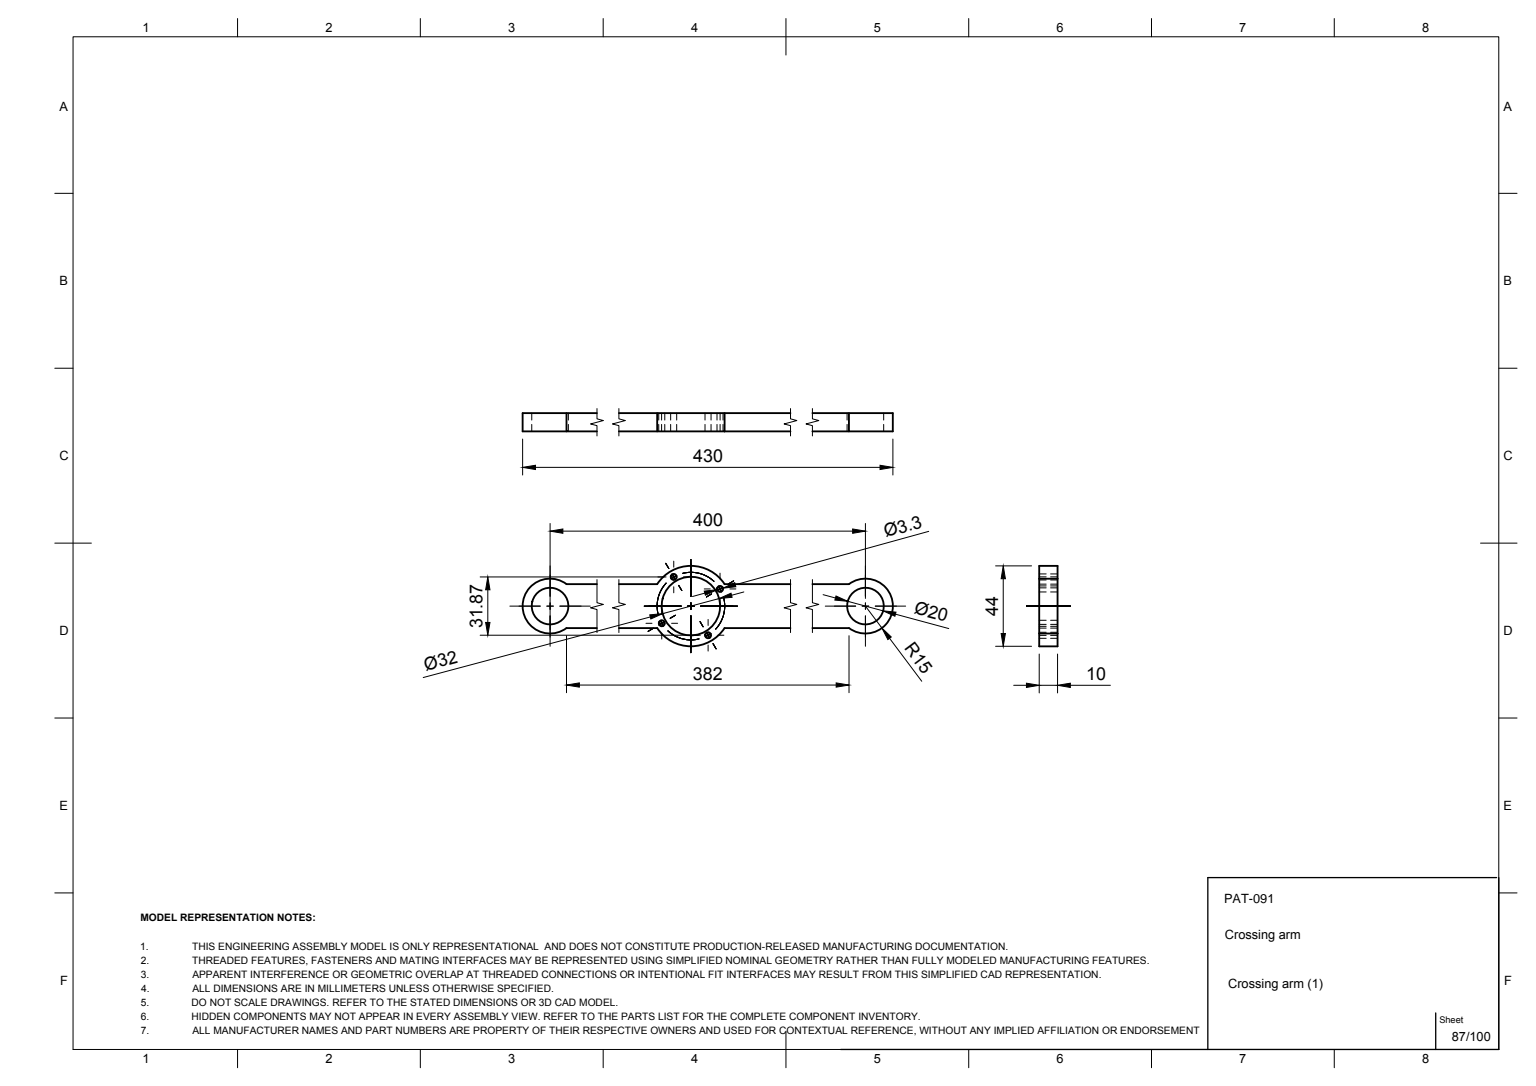
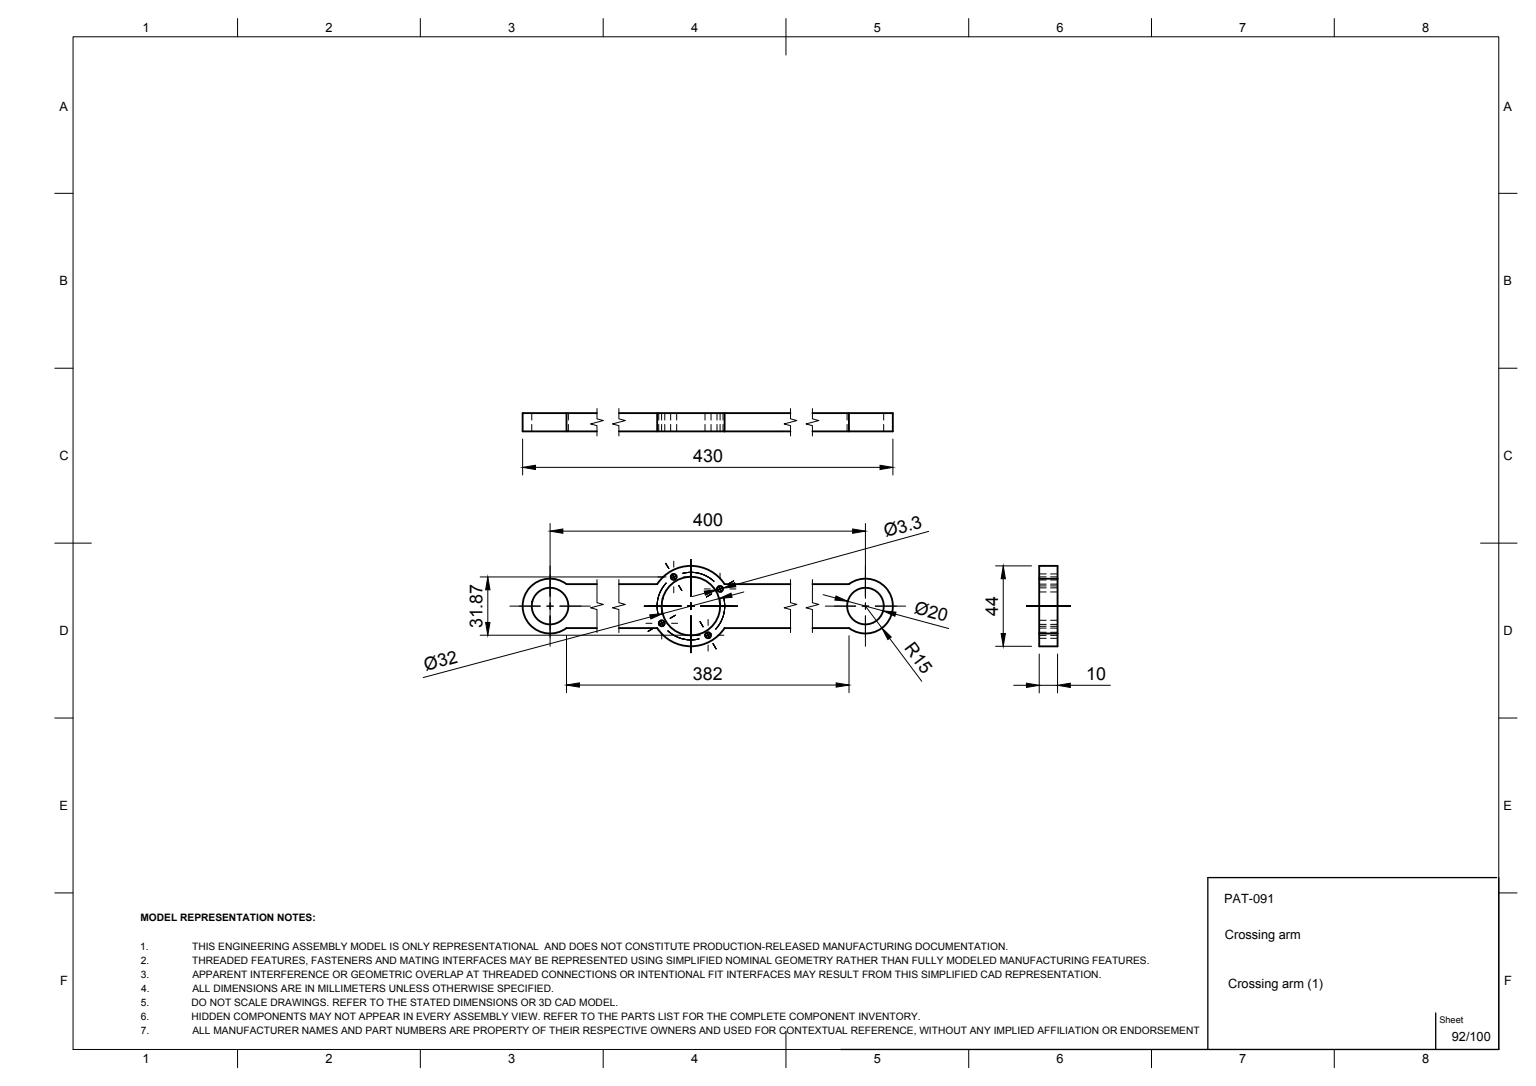
ISO-10303-21;
HEADER;
/* Generated by software containing ST-Developer
 * from STEP Tools, Inc. (www.steptools.com) 
 */

FILE_DESCRIPTION(
/* description */ ('PAT-091'),
/* implementation_level */ '2;1');

FILE_NAME(
/* name */ 'Crossing arm (1).step',
/* time_stamp */ '2026-10-27T15:34:44-07:00',
/* author */ (''),
/* organization */ (''),
/* preprocessor_version */ 'ST-DEVELOPER v20.2',
/* originating_system */ 'Autodesk Translation Framework v15.17.0.0',
/* authorisation */ '');

FILE_SCHEMA (('AUTOMOTIVE_DESIGN { 1 0 10303 214 3 1 1 }'));
ENDSEC;

DATA;
#10=MECHANICAL_DESIGN_GEOMETRIC_PRESENTATION_REPRESENTATION('',(#1057),#25100);
#837=SHAPE_REPRESENTATION_RELATIONSHIP('SRR','None',#25604,#947);
#947=ADVANCED_BREP_SHAPE_REPRESENTATION('',(#1178),#25074);
#1057=STYLED_ITEM('',(#26177),#1178);
#1178=MANIFOLD_SOLID_BREP('Body1',#13337);
#1571=FACE_BOUND('',#3877,.T.);
#1572=FACE_BOUND('',#3878,.T.);
#1573=FACE_BOUND('',#3879,.T.);
#1574=FACE_BOUND('',#3880,.T.);
#1575=FACE_BOUND('',#3881,.T.);
#1576=FACE_BOUND('',#3882,.T.);
#1577=FACE_BOUND('',#3883,.T.);
#1578=FACE_BOUND('',#3892,.T.);
#1579=FACE_BOUND('',#3893,.T.);
#1580=FACE_BOUND('',#3894,.T.);
#1581=FACE_BOUND('',#3895,.T.);
#1582=FACE_BOUND('',#3896,.T.);
#1583=FACE_BOUND('',#3897,.T.);
#1584=FACE_BOUND('',#3898,.T.);
#1986=PLANE('',#15974);
#1987=PLANE('',#15975);
#1988=PLANE('',#15980);
#1989=PLANE('',#15985);
#1990=PLANE('',#15990);
#1991=PLANE('',#15991);
#2694=FACE_OUTER_BOUND('',#3868,.T.);
#2695=FACE_OUTER_BOUND('',#3869,.T.);
#2696=FACE_OUTER_BOUND('',#3870,.T.);
#2697=FACE_OUTER_BOUND('',#3871,.T.);
#2698=FACE_OUTER_BOUND('',#3872,.T.);
#2699=FACE_OUTER_BOUND('',#3873,.T.);
#2700=FACE_OUTER_BOUND('',#3874,.T.);
#2701=FACE_OUTER_BOUND('',#3875,.T.);
#2702=FACE_OUTER_BOUND('',#3876,.T.);
#2703=FACE_OUTER_BOUND('',#3884,.T.);
#2704=FACE_OUTER_BOUND('',#3885,.T.);
#2705=FACE_OUTER_BOUND('',#3886,.T.);
#2706=FACE_OUTER_BOUND('',#3887,.T.);
#2707=FACE_OUTER_BOUND('',#3888,.T.);
#2708=FACE_OUTER_BOUND('',#3889,.T.);
#2709=FACE_OUTER_BOUND('',#3890,.T.);
#2710=FACE_OUTER_BOUND('',#3891,.T.);
#3868=EDGE_LOOP('',(#11426,#11427,#11428,#11429));
#3869=EDGE_LOOP('',(#11430,#11431,#11432,#11433));
#3870=EDGE_LOOP('',(#11434,#11435,#11436,#11437));
#3871=EDGE_LOOP('',(#11438,#11439,#11440,#11441));
#3872=EDGE_LOOP('',(#11442,#11443,#11444,#11445));
#3873=EDGE_LOOP('',(#11446,#11447,#11448,#11449));
#3874=EDGE_LOOP('',(#11450,#11451,#11452,#11453));
#3875=EDGE_LOOP('',(#11454,#11455,#11456,#11457));
#3876=EDGE_LOOP('',(#11458,#11459,#11460,#11461,#11462,#11463,#11464,#11465));
#3877=EDGE_LOOP('',(#11466));
#3878=EDGE_LOOP('',(#11467));
#3879=EDGE_LOOP('',(#11468));
#3880=EDGE_LOOP('',(#11469));
#3881=EDGE_LOOP('',(#11470));
#3882=EDGE_LOOP('',(#11471));
#3883=EDGE_LOOP('',(#11472));
#3884=EDGE_LOOP('',(#11473,#11474,#11475,#11476));
#3885=EDGE_LOOP('',(#11477,#11478,#11479,#11480));
#3886=EDGE_LOOP('',(#11481,#11482,#11483,#11484));
#3887=EDGE_LOOP('',(#11485,#11486,#11487,#11488));
#3888=EDGE_LOOP('',(#11489,#11490,#11491,#11492));
#3889=EDGE_LOOP('',(#11493,#11494,#11495,#11496));
#3890=EDGE_LOOP('',(#11497,#11498,#11499,#11500));
#3891=EDGE_LOOP('',(#11501,#11502,#11503,#11504,#11505,#11506,#11507,#11508));
#3892=EDGE_LOOP('',(#11509));
#3893=EDGE_LOOP('',(#11510));
#3894=EDGE_LOOP('',(#11511));
#3895=EDGE_LOOP('',(#11512));
#3896=EDGE_LOOP('',(#11513));
#3897=EDGE_LOOP('',(#11514));
#3898=EDGE_LOOP('',(#11515));
#4779=LINE('',#23871,#5519);
#4780=LINE('',#23877,#5520);
#4781=LINE('',#23883,#5521);
#4782=LINE('',#23889,#5522);
#4783=LINE('',#23895,#5523);
#4784=LINE('',#23900,#5524);
#4785=LINE('',#23904,#5525);
#4786=LINE('',#23909,#5526);
#4787=LINE('',#23913,#5527);
#4788=LINE('',#23917,#5528);
#4789=LINE('',#23919,#5529);
#4790=LINE('',#23920,#5530);
#4791=LINE('',#23924,#5531);
#4792=LINE('',#23926,#5532);
#4793=LINE('',#23929,#5533);
#4794=LINE('',#23936,#5534);
#4795=LINE('',#23937,#5535);
#4796=LINE('',#23941,#5536);
#4797=LINE('',#23944,#5537);
#4798=LINE('',#23947,#5538);
#4799=LINE('',#23949,#5539);
#4800=LINE('',#23953,#5540);
#4801=LINE('',#23957,#5541);
#5519=VECTOR('',#19863,0.164999999999999);
#5520=VECTOR('',#19870,0.164999999999999);
#5521=VECTOR('',#19877,0.164999999999999);
#5522=VECTOR('',#19884,0.164999999999999);
#5523=VECTOR('',#19891,1.6);
#5524=VECTOR('',#19896,1.);
#5525=VECTOR('',#19899,1.);
#5526=VECTOR('',#19904,1.);
#5527=VECTOR('',#19907,1.);
#5528=VECTOR('',#19912,1.);
#5529=VECTOR('',#19913,1.);
#5530=VECTOR('',#19914,1.);
#5531=VECTOR('',#19919,1.);
#5532=VECTOR('',#19920,1.);
#5533=VECTOR('',#19923,1.);
#5534=VECTOR('',#19930,1.);
#5535=VECTOR('',#19931,1.);
#5536=VECTOR('',#19936,1.);
#5537=VECTOR('',#19939,1.);
#5538=VECTOR('',#19942,1.);
#5539=VECTOR('',#19945,1.);
#5540=VECTOR('',#19950,1.);
#5541=VECTOR('',#19957,1.);
#6172=CIRCLE('',#15954,0.164999999999999);
#6173=CIRCLE('',#15955,0.164999999999999);
#6174=CIRCLE('',#15957,0.164999999999999);
#6175=CIRCLE('',#15958,0.164999999999999);
#6176=CIRCLE('',#15960,0.164999999999999);
#6177=CIRCLE('',#15961,0.164999999999999);
#6178=CIRCLE('',#15963,0.164999999999999);
#6179=CIRCLE('',#15964,0.164999999999999);
#6180=CIRCLE('',#15966,1.6);
#6181=CIRCLE('',#15967,1.6);
#6182=CIRCLE('',#15969,2.2);
#6183=CIRCLE('',#15970,2.2);
#6184=CIRCLE('',#15972,2.2);
#6185=CIRCLE('',#15973,2.2);
#6186=CIRCLE('',#15976,1.5);
#6187=CIRCLE('',#15977,1.5);
#6188=CIRCLE('',#15978,1.);
#6189=CIRCLE('',#15979,1.);
#6190=CIRCLE('',#15982,1.);
#6191=CIRCLE('',#15984,1.5);
#6192=CIRCLE('',#15987,1.);
#6193=CIRCLE('',#15989,1.5);
#7197=VERTEX_POINT('',#23868);
#7198=VERTEX_POINT('',#23870);
#7199=VERTEX_POINT('',#23874);
#7200=VERTEX_POINT('',#23876);
#7201=VERTEX_POINT('',#23880);
#7202=VERTEX_POINT('',#23882);
#7203=VERTEX_POINT('',#23886);
#7204=VERTEX_POINT('',#23888);
#7205=VERTEX_POINT('',#23892);
#7206=VERTEX_POINT('',#23894);
#7207=VERTEX_POINT('',#23898);
#7208=VERTEX_POINT('',#23899);
#7209=VERTEX_POINT('',#23901);
#7210=VERTEX_POINT('',#23903);
#7211=VERTEX_POINT('',#23907);
#7212=VERTEX_POINT('',#23908);
#7213=VERTEX_POINT('',#23910);
#7214=VERTEX_POINT('',#23912);
#7215=VERTEX_POINT('',#23916);
#7216=VERTEX_POINT('',#23918);
#7217=VERTEX_POINT('',#23922);
#7218=VERTEX_POINT('',#23925);
#7219=VERTEX_POINT('',#23927);
#7220=VERTEX_POINT('',#23930);
#7221=VERTEX_POINT('',#23932);
#7222=VERTEX_POINT('',#23935);
#7223=VERTEX_POINT('',#23939);
#7224=VERTEX_POINT('',#23943);
#7225=VERTEX_POINT('',#23945);
#7226=VERTEX_POINT('',#23951);
#8648=EDGE_CURVE('',#7197,#7197,#6172,.T.);
#8649=EDGE_CURVE('',#7197,#7198,#4779,.T.);
#8650=EDGE_CURVE('',#7198,#7198,#6173,.T.);
#8651=EDGE_CURVE('',#7199,#7199,#6174,.T.);
#8652=EDGE_CURVE('',#7199,#7200,#4780,.T.);
#8653=EDGE_CURVE('',#7200,#7200,#6175,.T.);
#8654=EDGE_CURVE('',#7201,#7201,#6176,.T.);
#8655=EDGE_CURVE('',#7201,#7202,#4781,.T.);
#8656=EDGE_CURVE('',#7202,#7202,#6177,.T.);
#8657=EDGE_CURVE('',#7203,#7203,#6178,.T.);
#8658=EDGE_CURVE('',#7203,#7204,#4782,.T.);
#8659=EDGE_CURVE('',#7204,#7204,#6179,.T.);
#8660=EDGE_CURVE('',#7205,#7205,#6180,.T.);
#8661=EDGE_CURVE('',#7205,#7206,#4783,.T.);
#8662=EDGE_CURVE('',#7206,#7206,#6181,.T.);
#8663=EDGE_CURVE('',#7207,#7208,#4784,.T.);
#8664=EDGE_CURVE('',#7209,#7207,#6182,.T.);
#8665=EDGE_CURVE('',#7210,#7209,#4785,.T.);
#8666=EDGE_CURVE('',#7210,#7208,#6183,.T.);
#8667=EDGE_CURVE('',#7211,#7212,#4786,.T.);
#8668=EDGE_CURVE('',#7211,#7213,#6184,.T.);
#8669=EDGE_CURVE('',#7214,#7213,#4787,.T.);
#8670=EDGE_CURVE('',#7212,#7214,#6185,.T.);
#8671=EDGE_CURVE('',#7213,#7215,#4788,.T.);
#8672=EDGE_CURVE('',#7215,#7216,#4789,.T.);
#8673=EDGE_CURVE('',#7214,#7216,#4790,.T.);
#8674=EDGE_CURVE('',#7216,#7217,#6186,.T.);
#8675=EDGE_CURVE('',#7217,#7209,#4791,.T.);
#8676=EDGE_CURVE('',#7207,#7218,#4792,.T.);
#8677=EDGE_CURVE('',#7218,#7219,#6187,.T.);
#8678=EDGE_CURVE('',#7219,#7212,#4793,.T.);
#8679=EDGE_CURVE('',#7220,#7220,#6188,.T.);
#8680=EDGE_CURVE('',#7221,#7221,#6189,.T.);
#8681=EDGE_CURVE('',#7217,#7222,#4794,.T.);
#8682=EDGE_CURVE('',#7222,#7210,#4795,.T.);
#8683=EDGE_CURVE('',#7223,#7223,#6190,.T.);
#8684=EDGE_CURVE('',#7223,#7220,#4796,.T.);
#8685=EDGE_CURVE('',#7224,#7218,#4797,.T.);
#8686=EDGE_CURVE('',#7224,#7225,#6191,.T.);
#8687=EDGE_CURVE('',#7219,#7225,#4798,.T.);
#8688=EDGE_CURVE('',#7208,#7224,#4799,.T.);
#8689=EDGE_CURVE('',#7226,#7226,#6192,.T.);
#8690=EDGE_CURVE('',#7226,#7221,#4800,.T.);
#8691=EDGE_CURVE('',#7215,#7222,#6193,.T.);
#8692=EDGE_CURVE('',#7225,#7211,#4801,.T.);
#11426=ORIENTED_EDGE('',*,*,#8648,.F.);
#11427=ORIENTED_EDGE('',*,*,#8649,.T.);
#11428=ORIENTED_EDGE('',*,*,#8650,.F.);
#11429=ORIENTED_EDGE('',*,*,#8649,.F.);
#11430=ORIENTED_EDGE('',*,*,#8651,.F.);
#11431=ORIENTED_EDGE('',*,*,#8652,.T.);
#11432=ORIENTED_EDGE('',*,*,#8653,.F.);
#11433=ORIENTED_EDGE('',*,*,#8652,.F.);
#11434=ORIENTED_EDGE('',*,*,#8654,.F.);
#11435=ORIENTED_EDGE('',*,*,#8655,.T.);
#11436=ORIENTED_EDGE('',*,*,#8656,.F.);
#11437=ORIENTED_EDGE('',*,*,#8655,.F.);
#11438=ORIENTED_EDGE('',*,*,#8657,.F.);
#11439=ORIENTED_EDGE('',*,*,#8658,.T.);
#11440=ORIENTED_EDGE('',*,*,#8659,.F.);
#11441=ORIENTED_EDGE('',*,*,#8658,.F.);
#11442=ORIENTED_EDGE('',*,*,#8660,.F.);
#11443=ORIENTED_EDGE('',*,*,#8661,.T.);
#11444=ORIENTED_EDGE('',*,*,#8662,.F.);
#11445=ORIENTED_EDGE('',*,*,#8661,.F.);
#11446=ORIENTED_EDGE('',*,*,#8663,.F.);
#11447=ORIENTED_EDGE('',*,*,#8664,.F.);
#11448=ORIENTED_EDGE('',*,*,#8665,.F.);
#11449=ORIENTED_EDGE('',*,*,#8666,.T.);
#11450=ORIENTED_EDGE('',*,*,#8667,.F.);
#11451=ORIENTED_EDGE('',*,*,#8668,.T.);
#11452=ORIENTED_EDGE('',*,*,#8669,.F.);
#11453=ORIENTED_EDGE('',*,*,#8670,.F.);
#11454=ORIENTED_EDGE('',*,*,#8669,.T.);
#11455=ORIENTED_EDGE('',*,*,#8671,.T.);
#11456=ORIENTED_EDGE('',*,*,#8672,.T.);
#11457=ORIENTED_EDGE('',*,*,#8673,.F.);
#11458=ORIENTED_EDGE('',*,*,#8673,.T.);
#11459=ORIENTED_EDGE('',*,*,#8674,.T.);
#11460=ORIENTED_EDGE('',*,*,#8675,.T.);
#11461=ORIENTED_EDGE('',*,*,#8664,.T.);
#11462=ORIENTED_EDGE('',*,*,#8676,.T.);
#11463=ORIENTED_EDGE('',*,*,#8677,.T.);
#11464=ORIENTED_EDGE('',*,*,#8678,.T.);
#11465=ORIENTED_EDGE('',*,*,#8670,.T.);
#11466=ORIENTED_EDGE('',*,*,#8679,.T.);
#11467=ORIENTED_EDGE('',*,*,#8680,.T.);
#11468=ORIENTED_EDGE('',*,*,#8662,.T.);
#11469=ORIENTED_EDGE('',*,*,#8659,.T.);
#11470=ORIENTED_EDGE('',*,*,#8656,.T.);
#11471=ORIENTED_EDGE('',*,*,#8653,.T.);
#11472=ORIENTED_EDGE('',*,*,#8650,.T.);
#11473=ORIENTED_EDGE('',*,*,#8665,.T.);
#11474=ORIENTED_EDGE('',*,*,#8675,.F.);
#11475=ORIENTED_EDGE('',*,*,#8681,.T.);
#11476=ORIENTED_EDGE('',*,*,#8682,.T.);
#11477=ORIENTED_EDGE('',*,*,#8683,.F.);
#11478=ORIENTED_EDGE('',*,*,#8684,.T.);
#11479=ORIENTED_EDGE('',*,*,#8679,.F.);
#11480=ORIENTED_EDGE('',*,*,#8684,.F.);
#11481=ORIENTED_EDGE('',*,*,#8685,.F.);
#11482=ORIENTED_EDGE('',*,*,#8686,.T.);
#11483=ORIENTED_EDGE('',*,*,#8687,.F.);
#11484=ORIENTED_EDGE('',*,*,#8677,.F.);
#11485=ORIENTED_EDGE('',*,*,#8663,.T.);
#11486=ORIENTED_EDGE('',*,*,#8688,.T.);
#11487=ORIENTED_EDGE('',*,*,#8685,.T.);
#11488=ORIENTED_EDGE('',*,*,#8676,.F.);
#11489=ORIENTED_EDGE('',*,*,#8689,.F.);
#11490=ORIENTED_EDGE('',*,*,#8690,.T.);
#11491=ORIENTED_EDGE('',*,*,#8680,.F.);
#11492=ORIENTED_EDGE('',*,*,#8690,.F.);
#11493=ORIENTED_EDGE('',*,*,#8672,.F.);
#11494=ORIENTED_EDGE('',*,*,#8691,.T.);
#11495=ORIENTED_EDGE('',*,*,#8681,.F.);
#11496=ORIENTED_EDGE('',*,*,#8674,.F.);
#11497=ORIENTED_EDGE('',*,*,#8667,.T.);
#11498=ORIENTED_EDGE('',*,*,#8678,.F.);
#11499=ORIENTED_EDGE('',*,*,#8687,.T.);
#11500=ORIENTED_EDGE('',*,*,#8692,.T.);
#11501=ORIENTED_EDGE('',*,*,#8692,.F.);
#11502=ORIENTED_EDGE('',*,*,#8686,.F.);
#11503=ORIENTED_EDGE('',*,*,#8688,.F.);
#11504=ORIENTED_EDGE('',*,*,#8666,.F.);
#11505=ORIENTED_EDGE('',*,*,#8682,.F.);
#11506=ORIENTED_EDGE('',*,*,#8691,.F.);
#11507=ORIENTED_EDGE('',*,*,#8671,.F.);
#11508=ORIENTED_EDGE('',*,*,#8668,.F.);
#11509=ORIENTED_EDGE('',*,*,#8683,.T.);
#11510=ORIENTED_EDGE('',*,*,#8689,.T.);
#11511=ORIENTED_EDGE('',*,*,#8660,.T.);
#11512=ORIENTED_EDGE('',*,*,#8657,.T.);
#11513=ORIENTED_EDGE('',*,*,#8654,.T.);
#11514=ORIENTED_EDGE('',*,*,#8651,.T.);
#11515=ORIENTED_EDGE('',*,*,#8648,.T.);
#12347=CYLINDRICAL_SURFACE('',#15953,0.164999999999999);
#12348=CYLINDRICAL_SURFACE('',#15956,0.164999999999999);
#12349=CYLINDRICAL_SURFACE('',#15959,0.164999999999999);
#12350=CYLINDRICAL_SURFACE('',#15962,0.164999999999999);
#12351=CYLINDRICAL_SURFACE('',#15965,1.6);
#12352=CYLINDRICAL_SURFACE('',#15968,2.2);
#12353=CYLINDRICAL_SURFACE('',#15971,2.2);
#12354=CYLINDRICAL_SURFACE('',#15981,1.);
#12355=CYLINDRICAL_SURFACE('',#15983,1.5);
#12356=CYLINDRICAL_SURFACE('',#15986,1.);
#12357=CYLINDRICAL_SURFACE('',#15988,1.5);
#13061=ADVANCED_FACE('',(#2694),#12347,.F.);
#13062=ADVANCED_FACE('',(#2695),#12348,.F.);
#13063=ADVANCED_FACE('',(#2696),#12349,.F.);
#13064=ADVANCED_FACE('',(#2697),#12350,.F.);
#13065=ADVANCED_FACE('',(#2698),#12351,.F.);
#13066=ADVANCED_FACE('',(#2699),#12352,.T.);
#13067=ADVANCED_FACE('',(#2700),#12353,.T.);
#13068=ADVANCED_FACE('',(#2701),#1986,.T.);
#13069=ADVANCED_FACE('',(#2702,#1571,#1572,#1573,#1574,#1575,#1576,#1577),
#1987,.T.);
#13070=ADVANCED_FACE('',(#2703),#1988,.T.);
#13071=ADVANCED_FACE('',(#2704),#12354,.F.);
#13072=ADVANCED_FACE('',(#2705),#12355,.T.);
#13073=ADVANCED_FACE('',(#2706),#1989,.T.);
#13074=ADVANCED_FACE('',(#2707),#12356,.F.);
#13075=ADVANCED_FACE('',(#2708),#12357,.T.);
#13076=ADVANCED_FACE('',(#2709),#1990,.T.);
#13077=ADVANCED_FACE('',(#2710,#1578,#1579,#1580,#1581,#1582,#1583,#1584),
#1991,.F.);
#13337=CLOSED_SHELL('',(#13061,#13062,#13063,#13064,#13065,#13066,#13067,
#13068,#13069,#13070,#13071,#13072,#13073,#13074,#13075,#13076,#13077));
#15952=AXIS2_PLACEMENT_3D('',#23866,#19857,#19858);
#15953=AXIS2_PLACEMENT_3D('',#23867,#19859,#19860);
#15954=AXIS2_PLACEMENT_3D('',#23869,#19861,#19862);
#15955=AXIS2_PLACEMENT_3D('',#23872,#19864,#19865);
#15956=AXIS2_PLACEMENT_3D('',#23873,#19866,#19867);
#15957=AXIS2_PLACEMENT_3D('',#23875,#19868,#19869);
#15958=AXIS2_PLACEMENT_3D('',#23878,#19871,#19872);
#15959=AXIS2_PLACEMENT_3D('',#23879,#19873,#19874);
#15960=AXIS2_PLACEMENT_3D('',#23881,#19875,#19876);
#15961=AXIS2_PLACEMENT_3D('',#23884,#19878,#19879);
#15962=AXIS2_PLACEMENT_3D('',#23885,#19880,#19881);
#15963=AXIS2_PLACEMENT_3D('',#23887,#19882,#19883);
#15964=AXIS2_PLACEMENT_3D('',#23890,#19885,#19886);
#15965=AXIS2_PLACEMENT_3D('',#23891,#19887,#19888);
#15966=AXIS2_PLACEMENT_3D('',#23893,#19889,#19890);
#15967=AXIS2_PLACEMENT_3D('',#23896,#19892,#19893);
#15968=AXIS2_PLACEMENT_3D('',#23897,#19894,#19895);
#15969=AXIS2_PLACEMENT_3D('',#23902,#19897,#19898);
#15970=AXIS2_PLACEMENT_3D('',#23905,#19900,#19901);
#15971=AXIS2_PLACEMENT_3D('',#23906,#19902,#19903);
#15972=AXIS2_PLACEMENT_3D('',#23911,#19905,#19906);
#15973=AXIS2_PLACEMENT_3D('',#23914,#19908,#19909);
#15974=AXIS2_PLACEMENT_3D('',#23915,#19910,#19911);
#15975=AXIS2_PLACEMENT_3D('',#23921,#19915,#19916);
#15976=AXIS2_PLACEMENT_3D('',#23923,#19917,#19918);
#15977=AXIS2_PLACEMENT_3D('',#23928,#19921,#19922);
#15978=AXIS2_PLACEMENT_3D('',#23931,#19924,#19925);
#15979=AXIS2_PLACEMENT_3D('',#23933,#19926,#19927);
#15980=AXIS2_PLACEMENT_3D('',#23934,#19928,#19929);
#15981=AXIS2_PLACEMENT_3D('',#23938,#19932,#19933);
#15982=AXIS2_PLACEMENT_3D('',#23940,#19934,#19935);
#15983=AXIS2_PLACEMENT_3D('',#23942,#19937,#19938);
#15984=AXIS2_PLACEMENT_3D('',#23946,#19940,#19941);
#15985=AXIS2_PLACEMENT_3D('',#23948,#19943,#19944);
#15986=AXIS2_PLACEMENT_3D('',#23950,#19946,#19947);
#15987=AXIS2_PLACEMENT_3D('',#23952,#19948,#19949);
#15988=AXIS2_PLACEMENT_3D('',#23954,#19951,#19952);
#15989=AXIS2_PLACEMENT_3D('',#23955,#19953,#19954);
#15990=AXIS2_PLACEMENT_3D('',#23956,#19955,#19956);
#15991=AXIS2_PLACEMENT_3D('',#23958,#19958,#19959);
#19857=DIRECTION('axis',(0.,0.,1.));
#19858=DIRECTION('refdir',(1.,0.,0.));
#19859=DIRECTION('center_axis',(0.,1.,0.));
#19860=DIRECTION('ref_axis',(1.,0.,0.));
#19861=DIRECTION('center_axis',(0.,1.,0.));
#19862=DIRECTION('ref_axis',(1.,0.,0.));
#19863=DIRECTION('',(0.,1.,0.));
#19864=DIRECTION('center_axis',(0.,-1.,0.));
#19865=DIRECTION('ref_axis',(1.,0.,0.));
#19866=DIRECTION('center_axis',(0.,1.,0.));
#19867=DIRECTION('ref_axis',(1.,0.,0.));
#19868=DIRECTION('center_axis',(0.,1.,0.));
#19869=DIRECTION('ref_axis',(1.,0.,0.));
#19870=DIRECTION('',(0.,1.,0.));
#19871=DIRECTION('center_axis',(0.,-1.,0.));
#19872=DIRECTION('ref_axis',(1.,0.,0.));
#19873=DIRECTION('center_axis',(0.,1.,0.));
#19874=DIRECTION('ref_axis',(1.,0.,0.));
#19875=DIRECTION('center_axis',(0.,1.,0.));
#19876=DIRECTION('ref_axis',(1.,0.,0.));
#19877=DIRECTION('',(0.,1.,0.));
#19878=DIRECTION('center_axis',(0.,-1.,0.));
#19879=DIRECTION('ref_axis',(1.,0.,0.));
#19880=DIRECTION('center_axis',(0.,1.,0.));
#19881=DIRECTION('ref_axis',(1.,0.,0.));
#19882=DIRECTION('center_axis',(0.,1.,0.));
#19883=DIRECTION('ref_axis',(1.,0.,0.));
#19884=DIRECTION('',(0.,1.,0.));
#19885=DIRECTION('center_axis',(0.,-1.,0.));
#19886=DIRECTION('ref_axis',(1.,0.,0.));
#19887=DIRECTION('center_axis',(0.,1.,0.));
#19888=DIRECTION('ref_axis',(1.,0.,0.));
#19889=DIRECTION('center_axis',(0.,1.,0.));
#19890=DIRECTION('ref_axis',(1.,0.,0.));
#19891=DIRECTION('',(0.,1.,0.));
#19892=DIRECTION('center_axis',(0.,-1.,0.));
#19893=DIRECTION('ref_axis',(1.,0.,0.));
#19894=DIRECTION('center_axis',(0.,1.,0.));
#19895=DIRECTION('ref_axis',(1.,0.,0.));
#19896=DIRECTION('',(0.,-1.,0.));
#19897=DIRECTION('center_axis',(0.,1.,0.));
#19898=DIRECTION('ref_axis',(1.,0.,0.));
#19899=DIRECTION('',(0.,1.,0.));
#19900=DIRECTION('center_axis',(0.,1.,0.));
#19901=DIRECTION('ref_axis',(1.,0.,0.));
#19902=DIRECTION('center_axis',(0.,1.,0.));
#19903=DIRECTION('ref_axis',(1.,0.,0.));
#19904=DIRECTION('',(0.,1.,0.));
#19905=DIRECTION('center_axis',(0.,1.,0.));
#19906=DIRECTION('ref_axis',(1.,0.,0.));
#19907=DIRECTION('',(0.,-1.,0.));
#19908=DIRECTION('center_axis',(0.,1.,0.));
#19909=DIRECTION('ref_axis',(1.,0.,0.));
#19910=DIRECTION('center_axis',(0.25,0.,0.968245836551854));
#19911=DIRECTION('ref_axis',(0.968245836551854,0.,-0.25));
#19912=DIRECTION('',(0.968245836551854,0.,-0.25));
#19913=DIRECTION('',(0.,1.,0.));
#19914=DIRECTION('',(0.968245836551854,0.,-0.25));
#19915=DIRECTION('center_axis',(0.,1.,0.));
#19916=DIRECTION('ref_axis',(0.,0.,1.));
#19917=DIRECTION('center_axis',(0.,1.,0.));
#19918=DIRECTION('ref_axis',(1.,0.,0.));
#19919=DIRECTION('',(-0.968245836551854,0.,0.25));
#19920=DIRECTION('',(-0.968245836551854,0.,0.25));
#19921=DIRECTION('center_axis',(0.,1.,0.));
#19922=DIRECTION('ref_axis',(1.,0.,0.));
#19923=DIRECTION('',(0.968245836551854,0.,-0.25));
#19924=DIRECTION('center_axis',(0.,-1.,0.));
#19925=DIRECTION('ref_axis',(1.,0.,0.));
#19926=DIRECTION('center_axis',(0.,-1.,0.));
#19927=DIRECTION('ref_axis',(1.,0.,0.));
#19928=DIRECTION('center_axis',(-0.25,0.,-0.968245836551854));
#19929=DIRECTION('ref_axis',(-0.968245836551854,0.,0.25));
#19930=DIRECTION('',(0.,-1.,0.));
#19931=DIRECTION('',(-0.968245836551854,0.,0.25));
#19932=DIRECTION('center_axis',(0.,1.,0.));
#19933=DIRECTION('ref_axis',(1.,0.,0.));
#19934=DIRECTION('center_axis',(0.,1.,0.));
#19935=DIRECTION('ref_axis',(1.,0.,0.));
#19936=DIRECTION('',(0.,1.,0.));
#19937=DIRECTION('center_axis',(0.,1.,0.));
#19938=DIRECTION('ref_axis',(-0.968245836551855,0.,0.249999999999998));
#19939=DIRECTION('',(0.,1.,0.));
#19940=DIRECTION('center_axis',(0.,1.,0.));
#19941=DIRECTION('ref_axis',(1.,0.,0.));
#19942=DIRECTION('',(0.,-1.,0.));
#19943=DIRECTION('center_axis',(-0.25,0.,-0.968245836551854));
#19944=DIRECTION('ref_axis',(-0.968245836551854,0.,0.25));
#19945=DIRECTION('',(-0.968245836551854,0.,0.25));
#19946=DIRECTION('center_axis',(0.,1.,0.));
#19947=DIRECTION('ref_axis',(1.,0.,0.));
#19948=DIRECTION('center_axis',(0.,1.,0.));
#19949=DIRECTION('ref_axis',(1.,0.,0.));
#19950=DIRECTION('',(0.,1.,0.));
#19951=DIRECTION('center_axis',(0.,1.,0.));
#19952=DIRECTION('ref_axis',(1.,0.,0.));
#19953=DIRECTION('center_axis',(0.,1.,0.));
#19954=DIRECTION('ref_axis',(1.,0.,0.));
#19955=DIRECTION('center_axis',(0.25,0.,0.968245836551854));
#19956=DIRECTION('ref_axis',(0.968245836551854,0.,-0.25));
#19957=DIRECTION('',(0.968245836551854,0.,-0.25));
#19958=DIRECTION('center_axis',(0.,1.,0.));
#19959=DIRECTION('ref_axis',(1.,0.,0.));
#23866=CARTESIAN_POINT('',(0.,0.,0.));
#23867=CARTESIAN_POINT('Origin',(18.056769185842,6.9,6.69185245480489));
#23868=CARTESIAN_POINT('',(17.891769185842,7.,6.69185245480489));
#23869=CARTESIAN_POINT('Origin',(18.056769185842,7.,6.69185245480489));
#23870=CARTESIAN_POINT('',(17.891769185842,8.,6.69185245480489));
#23871=CARTESIAN_POINT('',(17.891769185842,6.9,6.69185245480489));
#23872=CARTESIAN_POINT('Origin',(18.056769185842,8.,6.69185245480489));
#23873=CARTESIAN_POINT('Origin',(18.056769185842,6.9,9.30814754519511));
#23874=CARTESIAN_POINT('',(17.891769185842,7.,9.30814754519511));
#23875=CARTESIAN_POINT('Origin',(18.056769185842,7.,9.30814754519511));
#23876=CARTESIAN_POINT('',(17.891769185842,8.,9.30814754519511));
#23877=CARTESIAN_POINT('',(17.891769185842,6.9,9.30814754519511));
#23878=CARTESIAN_POINT('Origin',(18.056769185842,8.,9.30814754519511));
#23879=CARTESIAN_POINT('Origin',(20.6730642762322,6.9,9.30814754519511));
#23880=CARTESIAN_POINT('',(20.5080642762322,7.,9.30814754519511));
#23881=CARTESIAN_POINT('Origin',(20.6730642762322,7.,9.30814754519511));
#23882=CARTESIAN_POINT('',(20.5080642762322,8.,9.30814754519511));
#23883=CARTESIAN_POINT('',(20.5080642762322,6.9,9.30814754519511));
#23884=CARTESIAN_POINT('Origin',(20.6730642762322,8.,9.30814754519511));
#23885=CARTESIAN_POINT('Origin',(20.6730642762322,6.9,6.69185245480489));
#23886=CARTESIAN_POINT('',(20.5080642762322,7.,6.69185245480489));
#23887=CARTESIAN_POINT('Origin',(20.6730642762322,7.,6.69185245480489));
#23888=CARTESIAN_POINT('',(20.5080642762322,8.,6.69185245480489));
#23889=CARTESIAN_POINT('',(20.5080642762322,6.9,6.69185245480489));
#23890=CARTESIAN_POINT('Origin',(20.6730642762322,8.,6.69185245480489));
#23891=CARTESIAN_POINT('Origin',(19.3649167310371,6.9,8.));
#23892=CARTESIAN_POINT('',(17.7649167310371,7.,8.));
#23893=CARTESIAN_POINT('Origin',(19.3649167310371,7.,8.));
#23894=CARTESIAN_POINT('',(17.7649167310371,8.,8.));
#23895=CARTESIAN_POINT('',(17.7649167310371,6.9,8.));
#23896=CARTESIAN_POINT('Origin',(19.3649167310371,8.,8.));
#23897=CARTESIAN_POINT('Origin',(19.3649167310371,7.,8.));
#23898=CARTESIAN_POINT('',(17.2795596239014,8.,7.29908221900242));
#23899=CARTESIAN_POINT('',(17.2795596239014,7.,7.29908221900242));
#23900=CARTESIAN_POINT('',(17.2795596239014,7.,7.29908221900242));
#23901=CARTESIAN_POINT('',(20.8502738381728,8.,6.37712777327313));
#23902=CARTESIAN_POINT('Origin',(19.3649167310371,8.,8.));
#23903=CARTESIAN_POINT('',(20.8502738381728,7.,6.37712777327313));
#23904=CARTESIAN_POINT('',(20.8502738381728,7.,6.37712777327313));
#23905=CARTESIAN_POINT('Origin',(19.3649167310371,7.,8.));
#23906=CARTESIAN_POINT('Origin',(19.3649167310371,7.,8.));
#23907=CARTESIAN_POINT('',(17.8795596239014,7.,9.62287222672687));
#23908=CARTESIAN_POINT('',(17.8795596239014,8.,9.62287222672687));
#23909=CARTESIAN_POINT('',(17.8795596239014,7.,9.62287222672687));
#23910=CARTESIAN_POINT('',(21.4502738381728,7.,8.70091778099758));
#23911=CARTESIAN_POINT('Origin',(19.3649167310371,7.,8.));
#23912=CARTESIAN_POINT('',(21.4502738381728,8.,8.70091778099758));
#23913=CARTESIAN_POINT('',(21.4502738381728,7.,8.70091778099758));
#23914=CARTESIAN_POINT('Origin',(19.3649167310371,8.,8.));
#23915=CARTESIAN_POINT('Origin',(0.3,7.,14.1618950038622));
#23916=CARTESIAN_POINT('',(38.1584122091775,7.,4.38689500386223));
#23917=CARTESIAN_POINT('',(0.3,7.,14.1618950038622));
#23918=CARTESIAN_POINT('',(38.1584122091775,8.,4.38689500386223));
#23919=CARTESIAN_POINT('',(38.1584122091775,7.,4.38689500386223));
#23920=CARTESIAN_POINT('',(0.3,8.,14.1618950038622));
#23921=CARTESIAN_POINT('Origin',(19.3649167310371,8.,8.));
#23922=CARTESIAN_POINT('',(37.5584122091775,8.,2.06310499613778));
#23923=CARTESIAN_POINT('Origin',(38.7298334620742,8.,3.));
#23924=CARTESIAN_POINT('',(38.4298334620742,8.,1.83810499613777));
#23925=CARTESIAN_POINT('',(0.571421252896674,8.,11.6131049961378));
#23926=CARTESIAN_POINT('',(38.4298334620742,8.,1.83810499613777));
#23927=CARTESIAN_POINT('',(1.17142125289667,8.,13.9368950038622));
#23928=CARTESIAN_POINT('Origin',(0.,8.,13.));
#23929=CARTESIAN_POINT('',(0.3,8.,14.1618950038622));
#23930=CARTESIAN_POINT('',(-1.,8.,13.));
#23931=CARTESIAN_POINT('Origin',(0.,8.,13.));
#23932=CARTESIAN_POINT('',(37.7298334620742,8.,3.));
#23933=CARTESIAN_POINT('Origin',(38.7298334620742,8.,3.));
#23934=CARTESIAN_POINT('Origin',(38.4298334620742,7.,1.83810499613777));
#23935=CARTESIAN_POINT('',(37.5584122091775,7.,2.06310499613778));
#23936=CARTESIAN_POINT('',(37.5584122091775,7.,2.06310499613778));
#23937=CARTESIAN_POINT('',(38.4298334620742,7.,1.83810499613777));
#23938=CARTESIAN_POINT('Origin',(0.,6.9,13.));
#23939=CARTESIAN_POINT('',(-1.,7.,13.));
#23940=CARTESIAN_POINT('Origin',(0.,7.,13.));
#23941=CARTESIAN_POINT('',(-1.,6.9,13.));
#23942=CARTESIAN_POINT('Origin',(0.,7.,13.));
#23943=CARTESIAN_POINT('',(0.571421252896672,7.,11.6131049961378));
#23944=CARTESIAN_POINT('',(0.571421252896672,7.,11.6131049961378));
#23945=CARTESIAN_POINT('',(1.17142125289667,7.,13.9368950038622));
#23946=CARTESIAN_POINT('Origin',(0.,7.,13.));
#23947=CARTESIAN_POINT('',(1.17142125289667,7.,13.9368950038622));
#23948=CARTESIAN_POINT('Origin',(38.4298334620742,7.,1.83810499613777));
#23949=CARTESIAN_POINT('',(38.4298334620742,7.,1.83810499613777));
#23950=CARTESIAN_POINT('Origin',(38.7298334620742,6.9,3.));
#23951=CARTESIAN_POINT('',(37.7298334620742,7.,3.));
#23952=CARTESIAN_POINT('Origin',(38.7298334620742,7.,3.));
#23953=CARTESIAN_POINT('',(37.7298334620742,6.9,3.));
#23954=CARTESIAN_POINT('Origin',(38.7298334620742,7.,3.));
#23955=CARTESIAN_POINT('Origin',(38.7298334620742,7.,3.));
#23956=CARTESIAN_POINT('Origin',(0.3,7.,14.1618950038622));
#23957=CARTESIAN_POINT('',(0.3,7.,14.1618950038622));
#23958=CARTESIAN_POINT('Origin',(19.3649167310371,7.,8.));
#24953=UNCERTAINTY_MEASURE_WITH_UNIT(LENGTH_MEASURE(0.001),#25101,
'DISTANCE_ACCURACY_VALUE',
'Maximum model space distance between geometric entities at asserted c
onnectivities');
#24979=UNCERTAINTY_MEASURE_WITH_UNIT(LENGTH_MEASURE(0.001),#25101,
'DISTANCE_ACCURACY_VALUE',
'Maximum model space distance between geometric entities at asserted c
onnectivities');
#25074=(
GEOMETRIC_REPRESENTATION_CONTEXT(3)
GLOBAL_UNCERTAINTY_ASSIGNED_CONTEXT((#24953))
GLOBAL_UNIT_ASSIGNED_CONTEXT((#25101,#25103,#25104))
REPRESENTATION_CONTEXT('','3D')
);
#25100=(
GEOMETRIC_REPRESENTATION_CONTEXT(3)
GLOBAL_UNCERTAINTY_ASSIGNED_CONTEXT((#24979))
GLOBAL_UNIT_ASSIGNED_CONTEXT((#25101,#25103,#25104))
REPRESENTATION_CONTEXT('','3D')
);
#25101=(
LENGTH_UNIT()
NAMED_UNIT(*)
SI_UNIT(.CENTI.,.METRE.)
);
#25103=(
NAMED_UNIT(*)
PLANE_ANGLE_UNIT()
SI_UNIT($,.RADIAN.)
);
#25104=(
NAMED_UNIT(*)
SI_UNIT($,.STERADIAN.)
SOLID_ANGLE_UNIT()
);
#25199=SHAPE_DEFINITION_REPRESENTATION(#25393,#25604);
#25393=PRODUCT_DEFINITION_SHAPE('',$,#25725);
#25604=SHAPE_REPRESENTATION('',(#15952),#25074);
#25630=PRODUCT_DEFINITION_CONTEXT('part definition',#25992,'design');
#25725=PRODUCT_DEFINITION('Crossing arm (1)','Crossing arm (1)',#25845,#25630);
#25845=PRODUCT_DEFINITION_FORMATION('',$,#26088);
#25992=APPLICATION_CONTEXT(
'Core Data for Automotive Mechanical Design Process');
#25993=PRODUCT_CONTEXT('part definition',#25992,'mechanical');
#26088=PRODUCT('Crossing arm (1)','Crossing arm (1)','Crossing arm (1)',(#25993));
#26171=COLOUR_RGB('Light Blue',0.38,0.62,0.78);
#26172=FILL_AREA_STYLE_COLOUR('',#26171);
#26173=FILL_AREA_STYLE('',(#26172));
#26174=SURFACE_STYLE_FILL_AREA(#26173);
#26175=SURFACE_SIDE_STYLE('',(#26174));
#26176=SURFACE_STYLE_USAGE(.BOTH.,#26175);
#26177=PRESENTATION_STYLE_ASSIGNMENT((#26176));
ENDSEC;
END-ISO-10303-21;
